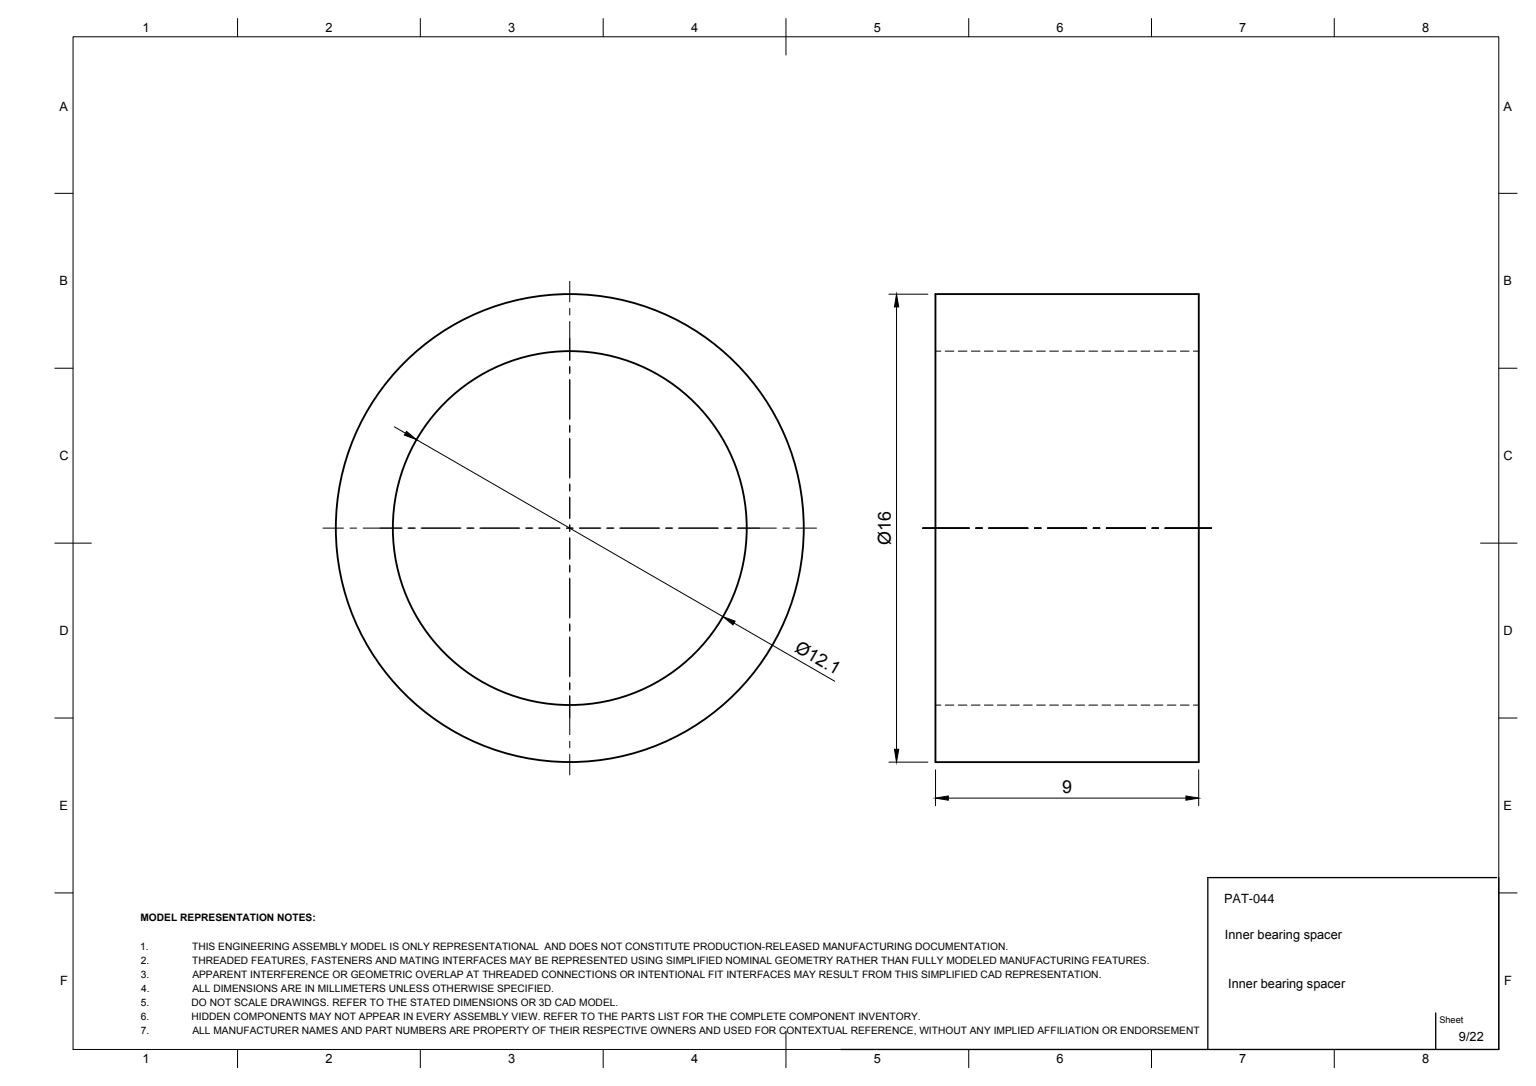
ISO-10303-21;
HEADER;
/* Generated by software containing ST-Developer
 * from STEP Tools, Inc. (www.steptools.com) 
 */

FILE_DESCRIPTION(
/* description */ ('Four-wheel beam trolley'),
/* implementation_level */ '2;1');

FILE_NAME(
/* name */ 'Inner bearing spacer.step',
/* time_stamp */ '2026-10-29T16:22:06-07:00',
/* author */ (''),
/* organization */ (''),
/* preprocessor_version */ 'ST-DEVELOPER v20.2',
/* originating_system */ 'Autodesk Translation Framework v15.17.0.0',
/* authorisation */ '');

FILE_SCHEMA (('AUTOMOTIVE_DESIGN { 1 0 10303 214 3 1 1 }'));
ENDSEC;

DATA;
#10=MECHANICAL_DESIGN_GEOMETRIC_PRESENTATION_REPRESENTATION('',(#284),#4777);
#250=SHAPE_REPRESENTATION_RELATIONSHIP('SRR','None',#4879,#267);
#267=ADVANCED_BREP_SHAPE_REPRESENTATION('',(#307),#4764);
#284=STYLED_ITEM('',(#5056),#307);
#307=MANIFOLD_SOLID_BREP('Body1',#2372);
#343=FACE_BOUND('',#670,.T.);
#344=FACE_BOUND('',#672,.T.);
#403=PLANE('',#2691);
#404=PLANE('',#2692);
#501=FACE_OUTER_BOUND('',#667,.T.);
#502=FACE_OUTER_BOUND('',#668,.T.);
#503=FACE_OUTER_BOUND('',#669,.T.);
#504=FACE_OUTER_BOUND('',#671,.T.);
#667=EDGE_LOOP('',(#1845,#1846,#1847,#1848));
#668=EDGE_LOOP('',(#1849,#1850,#1851,#1852));
#669=EDGE_LOOP('',(#1853));
#670=EDGE_LOOP('',(#1854));
#671=EDGE_LOOP('',(#1855));
#672=EDGE_LOOP('',(#1856));
#849=LINE('',#4015,#972);
#850=LINE('',#4021,#973);
#972=VECTOR('',#3220,0.605);
#973=VECTOR('',#3227,0.8);
#1061=CIRCLE('',#2686,0.605);
#1062=CIRCLE('',#2687,0.605);
#1063=CIRCLE('',#2689,0.8);
#1064=CIRCLE('',#2690,0.8);
#1233=VERTEX_POINT('',#4012);
#1234=VERTEX_POINT('',#4014);
#1235=VERTEX_POINT('',#4018);
#1236=VERTEX_POINT('',#4020);
#1460=EDGE_CURVE('',#1233,#1233,#1061,.T.);
#1461=EDGE_CURVE('',#1233,#1234,#849,.T.);
#1462=EDGE_CURVE('',#1234,#1234,#1062,.T.);
#1463=EDGE_CURVE('',#1235,#1235,#1063,.T.);
#1464=EDGE_CURVE('',#1235,#1236,#850,.T.);
#1465=EDGE_CURVE('',#1236,#1236,#1064,.T.);
#1845=ORIENTED_EDGE('',*,*,#1460,.F.);
#1846=ORIENTED_EDGE('',*,*,#1461,.T.);
#1847=ORIENTED_EDGE('',*,*,#1462,.T.);
#1848=ORIENTED_EDGE('',*,*,#1461,.F.);
#1849=ORIENTED_EDGE('',*,*,#1463,.F.);
#1850=ORIENTED_EDGE('',*,*,#1464,.T.);
#1851=ORIENTED_EDGE('',*,*,#1465,.T.);
#1852=ORIENTED_EDGE('',*,*,#1464,.F.);
#1853=ORIENTED_EDGE('',*,*,#1463,.T.);
#1854=ORIENTED_EDGE('',*,*,#1460,.T.);
#1855=ORIENTED_EDGE('',*,*,#1465,.F.);
#1856=ORIENTED_EDGE('',*,*,#1462,.F.);
#2192=CYLINDRICAL_SURFACE('',#2685,0.605);
#2193=CYLINDRICAL_SURFACE('',#2688,0.8);
#2277=ADVANCED_FACE('',(#501),#2192,.F.);
#2278=ADVANCED_FACE('',(#502),#2193,.T.);
#2279=ADVANCED_FACE('',(#503,#343),#403,.T.);
#2280=ADVANCED_FACE('',(#504,#344),#404,.F.);
#2372=CLOSED_SHELL('',(#2277,#2278,#2279,#2280));
#2684=AXIS2_PLACEMENT_3D('',#4010,#3214,#3215);
#2685=AXIS2_PLACEMENT_3D('',#4011,#3216,#3217);
#2686=AXIS2_PLACEMENT_3D('',#4013,#3218,#3219);
#2687=AXIS2_PLACEMENT_3D('',#4016,#3221,#3222);
#2688=AXIS2_PLACEMENT_3D('',#4017,#3223,#3224);
#2689=AXIS2_PLACEMENT_3D('',#4019,#3225,#3226);
#2690=AXIS2_PLACEMENT_3D('',#4022,#3228,#3229);
#2691=AXIS2_PLACEMENT_3D('',#4023,#3230,#3231);
#2692=AXIS2_PLACEMENT_3D('',#4024,#3232,#3233);
#3214=DIRECTION('axis',(0.,0.,1.));
#3215=DIRECTION('refdir',(1.,0.,0.));
#3216=DIRECTION('center_axis',(0.,1.,0.));
#3217=DIRECTION('ref_axis',(1.,0.,0.));
#3218=DIRECTION('center_axis',(0.,-1.,0.));
#3219=DIRECTION('ref_axis',(1.,0.,0.));
#3220=DIRECTION('',(0.,-1.,0.));
#3221=DIRECTION('center_axis',(0.,-1.,0.));
#3222=DIRECTION('ref_axis',(1.,0.,0.));
#3223=DIRECTION('center_axis',(0.,1.,0.));
#3224=DIRECTION('ref_axis',(1.,0.,0.));
#3225=DIRECTION('center_axis',(0.,1.,0.));
#3226=DIRECTION('ref_axis',(1.,0.,0.));
#3227=DIRECTION('',(0.,-1.,0.));
#3228=DIRECTION('center_axis',(0.,1.,0.));
#3229=DIRECTION('ref_axis',(1.,0.,0.));
#3230=DIRECTION('center_axis',(0.,1.,0.));
#3231=DIRECTION('ref_axis',(1.,0.,0.));
#3232=DIRECTION('center_axis',(0.,1.,0.));
#3233=DIRECTION('ref_axis',(1.,0.,0.));
#4010=CARTESIAN_POINT('',(0.,0.,0.));
#4011=CARTESIAN_POINT('Origin',(0.,1.,13.75));
#4012=CARTESIAN_POINT('',(-0.605,1.9,13.75));
#4013=CARTESIAN_POINT('Origin',(0.,1.9,13.75));
#4014=CARTESIAN_POINT('',(-0.605,1.,13.75));
#4015=CARTESIAN_POINT('',(-0.605,1.,13.75));
#4016=CARTESIAN_POINT('Origin',(0.,1.,13.75));
#4017=CARTESIAN_POINT('Origin',(0.,1.,13.75));
#4018=CARTESIAN_POINT('',(-0.8,1.9,13.75));
#4019=CARTESIAN_POINT('Origin',(0.,1.9,13.75));
#4020=CARTESIAN_POINT('',(-0.8,1.,13.75));
#4021=CARTESIAN_POINT('',(-0.8,1.,13.75));
#4022=CARTESIAN_POINT('Origin',(0.,1.,13.75));
#4023=CARTESIAN_POINT('Origin',(0.,1.9,13.75));
#4024=CARTESIAN_POINT('Origin',(0.,1.,13.75));
#4742=UNCERTAINTY_MEASURE_WITH_UNIT(LENGTH_MEASURE(0.001),#4778,
'DISTANCE_ACCURACY_VALUE',
'Maximum model space distance between geometric entities at asserted c
onnectivities');
#4755=UNCERTAINTY_MEASURE_WITH_UNIT(LENGTH_MEASURE(0.001),#4778,
'DISTANCE_ACCURACY_VALUE',
'Maximum model space distance between geometric entities at asserted c
onnectivities');
#4764=(
GEOMETRIC_REPRESENTATION_CONTEXT(3)
GLOBAL_UNCERTAINTY_ASSIGNED_CONTEXT((#4742))
GLOBAL_UNIT_ASSIGNED_CONTEXT((#4778,#4780,#4781))
REPRESENTATION_CONTEXT('','3D')
);
#4777=(
GEOMETRIC_REPRESENTATION_CONTEXT(3)
GLOBAL_UNCERTAINTY_ASSIGNED_CONTEXT((#4755))
GLOBAL_UNIT_ASSIGNED_CONTEXT((#4778,#4780,#4781))
REPRESENTATION_CONTEXT('','3D')
);
#4778=(
LENGTH_UNIT()
NAMED_UNIT(*)
SI_UNIT(.CENTI.,.METRE.)
);
#4780=(
NAMED_UNIT(*)
PLANE_ANGLE_UNIT()
SI_UNIT($,.RADIAN.)
);
#4781=(
NAMED_UNIT(*)
SI_UNIT($,.STERADIAN.)
SOLID_ANGLE_UNIT()
);
#4790=SHAPE_DEFINITION_REPRESENTATION(#4811,#4879);
#4811=PRODUCT_DEFINITION_SHAPE('',$,#4901);
#4879=SHAPE_REPRESENTATION('',(#2684),#4764);
#4892=PRODUCT_DEFINITION_CONTEXT('part definition',#4957,'design');
#4901=PRODUCT_DEFINITION('Inner bearing spacer','Inner bearing spacer',
#4922,#4892);
#4922=PRODUCT_DEFINITION_FORMATION('',$,#4967);
#4957=APPLICATION_CONTEXT(
'Core Data for Automotive Mechanical Design Process');
#4958=PRODUCT_CONTEXT('part definition',#4957,'mechanical');
#4967=PRODUCT('Inner bearing spacer','Inner bearing spacer',
'Inner bearing spacer',(#4958));
#5050=COLOUR_RGB('Grey',0.48,0.52,0.57);
#5051=FILL_AREA_STYLE_COLOUR('',#5050);
#5052=FILL_AREA_STYLE('',(#5051));
#5053=SURFACE_STYLE_FILL_AREA(#5052);
#5054=SURFACE_SIDE_STYLE('',(#5053));
#5055=SURFACE_STYLE_USAGE(.BOTH.,#5054);
#5056=PRESENTATION_STYLE_ASSIGNMENT((#5055));
ENDSEC;
END-ISO-10303-21;
